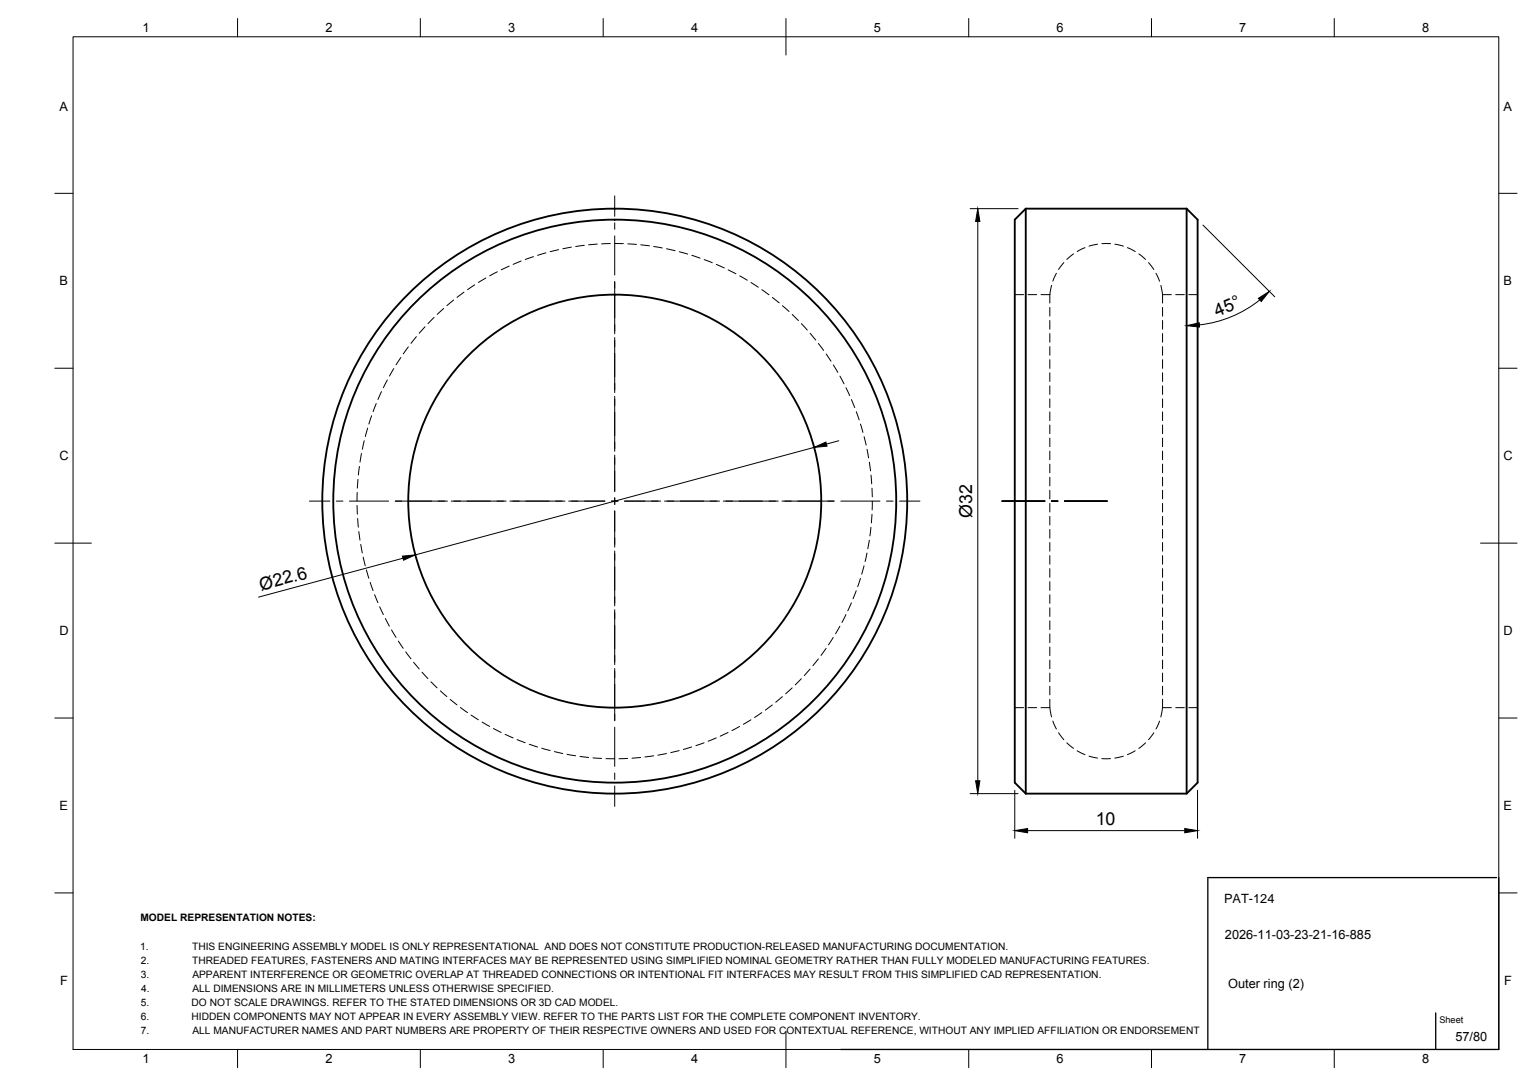
ISO-10303-21;
HEADER;
/* Generated by software containing ST-Developer
 * from STEP Tools, Inc. (www.steptools.com) 
 */

FILE_DESCRIPTION(
/* description */ ('XY cross-slide table'),
/* implementation_level */ '2;1');

FILE_NAME(
/* name */ 'Outer ring (2).step',
/* time_stamp */ '2026-10-28T03:22:46-07:00',
/* author */ (''),
/* organization */ (''),
/* preprocessor_version */ 'ST-DEVELOPER v20.2',
/* originating_system */ 'Autodesk Translation Framework v15.17.0.0',
/* authorisation */ '');

FILE_SCHEMA (('AUTOMOTIVE_DESIGN { 1 0 10303 214 3 1 1 }'));
ENDSEC;

DATA;
#10=MECHANICAL_DESIGN_GEOMETRIC_PRESENTATION_REPRESENTATION('',(#1737),#62984);
#1469=CONICAL_SURFACE('',#25563,1.57,0.785398163397449);
#1470=CONICAL_SURFACE('',#25567,1.57,0.785398163397449);
#1501=TOROIDAL_SURFACE('',#25552,1.1,0.309556);
#1556=SHAPE_REPRESENTATION_RELATIONSHIP('SRR','None',#63412,#1639);
#1639=ADVANCED_BREP_SHAPE_REPRESENTATION('',(#1846),#62949);
#1737=STYLED_ITEM('',(#63912),#1846);
#1846=MANIFOLD_SOLID_BREP('Body1',#23035);
#2203=FACE_BOUND('',#5316,.T.);
#2204=FACE_BOUND('',#5321,.T.);
#2664=PLANE('',#25560);
#2665=PLANE('',#25569);
#3683=FACE_OUTER_BOUND('',#5313,.T.);
#3684=FACE_OUTER_BOUND('',#5314,.T.);
#3685=FACE_OUTER_BOUND('',#5315,.T.);
#3686=FACE_OUTER_BOUND('',#5317,.T.);
#3687=FACE_OUTER_BOUND('',#5318,.T.);
#3688=FACE_OUTER_BOUND('',#5319,.T.);
#3689=FACE_OUTER_BOUND('',#5320,.T.);
#3690=FACE_OUTER_BOUND('',#5322,.T.);
#5313=EDGE_LOOP('',(#18660,#18661,#18662,#18663,#18664,#18665));
#5314=EDGE_LOOP('',(#18666,#18667,#18668,#18669,#18670));
#5315=EDGE_LOOP('',(#18671));
#5316=EDGE_LOOP('',(#18672));
#5317=EDGE_LOOP('',(#18673,#18674,#18675,#18676));
#5318=EDGE_LOOP('',(#18677,#18678,#18679,#18680));
#5319=EDGE_LOOP('',(#18681,#18682,#18683,#18684));
#5320=EDGE_LOOP('',(#18685));
#5321=EDGE_LOOP('',(#18686));
#5322=EDGE_LOOP('',(#18687,#18688,#18689,#18690,#18691));
#6842=LINE('',#48582,#8329);
#6843=LINE('',#48591,#8330);
#6844=LINE('',#48595,#8331);
#6845=LINE('',#48599,#8332);
#6846=LINE('',#48602,#8333);
#8329=VECTOR('',#30517,1.129765);
#8330=VECTOR('',#30528,1.57);
#8331=VECTOR('',#30533,1.6);
#8332=VECTOR('',#30538,1.57);
#8333=VECTOR('',#30543,1.129765);
#9478=CIRCLE('',#25553,1.129765);
#9479=CIRCLE('',#25554,1.129765);
#9480=CIRCLE('',#25555,0.309556);
#9481=CIRCLE('',#25556,1.129765);
#9482=CIRCLE('',#25557,1.129765);
#9483=CIRCLE('',#25559,1.129765);
#9484=CIRCLE('',#25561,1.54);
#9485=CIRCLE('',#25562,1.129765);
#9486=CIRCLE('',#25564,1.6);
#9487=CIRCLE('',#25566,1.6);
#9488=CIRCLE('',#25568,1.54);
#11031=VERTEX_POINT('',#48570);
#11032=VERTEX_POINT('',#48571);
#11033=VERTEX_POINT('',#48574);
#11034=VERTEX_POINT('',#48576);
#11035=VERTEX_POINT('',#48580);
#11036=VERTEX_POINT('',#48584);
#11037=VERTEX_POINT('',#48586);
#11038=VERTEX_POINT('',#48589);
#11039=VERTEX_POINT('',#48593);
#11040=VERTEX_POINT('',#48597);
#13714=EDGE_CURVE('',#11031,#11032,#9478,.T.);
#13715=EDGE_CURVE('',#11032,#11031,#9479,.T.);
#13716=EDGE_CURVE('',#11032,#11033,#9480,.T.);
#13717=EDGE_CURVE('',#11034,#11033,#9481,.T.);
#13718=EDGE_CURVE('',#11033,#11034,#9482,.T.);
#13719=EDGE_CURVE('',#11035,#11035,#9483,.T.);
#13720=EDGE_CURVE('',#11035,#11034,#6842,.T.);
#13721=EDGE_CURVE('',#11036,#11036,#9484,.T.);
#13722=EDGE_CURVE('',#11037,#11037,#9485,.T.);
#13723=EDGE_CURVE('',#11038,#11038,#9486,.T.);
#13724=EDGE_CURVE('',#11038,#11036,#6843,.T.);
#13725=EDGE_CURVE('',#11039,#11039,#9487,.T.);
#13726=EDGE_CURVE('',#11039,#11038,#6844,.T.);
#13727=EDGE_CURVE('',#11040,#11040,#9488,.T.);
#13728=EDGE_CURVE('',#11040,#11039,#6845,.T.);
#13729=EDGE_CURVE('',#11031,#11037,#6846,.T.);
#18660=ORIENTED_EDGE('',*,*,#13714,.F.);
#18661=ORIENTED_EDGE('',*,*,#13715,.F.);
#18662=ORIENTED_EDGE('',*,*,#13716,.T.);
#18663=ORIENTED_EDGE('',*,*,#13717,.F.);
#18664=ORIENTED_EDGE('',*,*,#13718,.F.);
#18665=ORIENTED_EDGE('',*,*,#13716,.F.);
#18666=ORIENTED_EDGE('',*,*,#13719,.T.);
#18667=ORIENTED_EDGE('',*,*,#13720,.T.);
#18668=ORIENTED_EDGE('',*,*,#13717,.T.);
#18669=ORIENTED_EDGE('',*,*,#13718,.T.);
#18670=ORIENTED_EDGE('',*,*,#13720,.F.);
#18671=ORIENTED_EDGE('',*,*,#13721,.F.);
#18672=ORIENTED_EDGE('',*,*,#13722,.T.);
#18673=ORIENTED_EDGE('',*,*,#13723,.F.);
#18674=ORIENTED_EDGE('',*,*,#13724,.T.);
#18675=ORIENTED_EDGE('',*,*,#13721,.T.);
#18676=ORIENTED_EDGE('',*,*,#13724,.F.);
#18677=ORIENTED_EDGE('',*,*,#13725,.F.);
#18678=ORIENTED_EDGE('',*,*,#13726,.T.);
#18679=ORIENTED_EDGE('',*,*,#13723,.T.);
#18680=ORIENTED_EDGE('',*,*,#13726,.F.);
#18681=ORIENTED_EDGE('',*,*,#13727,.F.);
#18682=ORIENTED_EDGE('',*,*,#13728,.T.);
#18683=ORIENTED_EDGE('',*,*,#13725,.T.);
#18684=ORIENTED_EDGE('',*,*,#13728,.F.);
#18685=ORIENTED_EDGE('',*,*,#13727,.T.);
#18686=ORIENTED_EDGE('',*,*,#13719,.F.);
#18687=ORIENTED_EDGE('',*,*,#13714,.T.);
#18688=ORIENTED_EDGE('',*,*,#13715,.T.);
#18689=ORIENTED_EDGE('',*,*,#13729,.T.);
#18690=ORIENTED_EDGE('',*,*,#13722,.F.);
#18691=ORIENTED_EDGE('',*,*,#13729,.F.);
#21419=CYLINDRICAL_SURFACE('',#25558,1.129765);
#21420=CYLINDRICAL_SURFACE('',#25565,1.6);
#21421=CYLINDRICAL_SURFACE('',#25570,1.129765);
#22464=ADVANCED_FACE('',(#3683),#1501,.F.);
#22465=ADVANCED_FACE('',(#3684),#21419,.F.);
#22466=ADVANCED_FACE('',(#3685,#2203),#2664,.T.);
#22467=ADVANCED_FACE('',(#3686),#1469,.T.);
#22468=ADVANCED_FACE('',(#3687),#21420,.T.);
#22469=ADVANCED_FACE('',(#3688),#1470,.T.);
#22470=ADVANCED_FACE('',(#3689,#2204),#2665,.T.);
#22471=ADVANCED_FACE('',(#3690),#21421,.F.);
#23035=CLOSED_SHELL('',(#22464,#22465,#22466,#22467,#22468,#22469,#22470,
#22471));
#25551=AXIS2_PLACEMENT_3D('',#48568,#30499,#30500);
#25552=AXIS2_PLACEMENT_3D('',#48569,#30501,#30502);
#25553=AXIS2_PLACEMENT_3D('',#48572,#30503,#30504);
#25554=AXIS2_PLACEMENT_3D('',#48573,#30505,#30506);
#25555=AXIS2_PLACEMENT_3D('',#48575,#30507,#30508);
#25556=AXIS2_PLACEMENT_3D('',#48577,#30509,#30510);
#25557=AXIS2_PLACEMENT_3D('',#48578,#30511,#30512);
#25558=AXIS2_PLACEMENT_3D('',#48579,#30513,#30514);
#25559=AXIS2_PLACEMENT_3D('',#48581,#30515,#30516);
#25560=AXIS2_PLACEMENT_3D('',#48583,#30518,#30519);
#25561=AXIS2_PLACEMENT_3D('',#48585,#30520,#30521);
#25562=AXIS2_PLACEMENT_3D('',#48587,#30522,#30523);
#25563=AXIS2_PLACEMENT_3D('',#48588,#30524,#30525);
#25564=AXIS2_PLACEMENT_3D('',#48590,#30526,#30527);
#25565=AXIS2_PLACEMENT_3D('',#48592,#30529,#30530);
#25566=AXIS2_PLACEMENT_3D('',#48594,#30531,#30532);
#25567=AXIS2_PLACEMENT_3D('',#48596,#30534,#30535);
#25568=AXIS2_PLACEMENT_3D('',#48598,#30536,#30537);
#25569=AXIS2_PLACEMENT_3D('',#48600,#30539,#30540);
#25570=AXIS2_PLACEMENT_3D('',#48601,#30541,#30542);
#30499=DIRECTION('axis',(0.,0.,1.));
#30500=DIRECTION('refdir',(1.,0.,0.));
#30501=DIRECTION('center_axis',(0.,-1.,0.));
#30502=DIRECTION('ref_axis',(0.,0.,-1.));
#30503=DIRECTION('center_axis',(0.,-1.,0.));
#30504=DIRECTION('ref_axis',(1.,0.,0.));
#30505=DIRECTION('center_axis',(0.,-1.,0.));
#30506=DIRECTION('ref_axis',(1.,0.,0.));
#30507=DIRECTION('center_axis',(1.,0.,1.22464679914735E-16));
#30508=DIRECTION('ref_axis',(-1.22464679914735E-16,0.,1.));
#30509=DIRECTION('center_axis',(0.,1.,0.));
#30510=DIRECTION('ref_axis',(1.,0.,0.));
#30511=DIRECTION('center_axis',(0.,1.,0.));
#30512=DIRECTION('ref_axis',(1.,0.,0.));
#30513=DIRECTION('center_axis',(0.,-1.,0.));
#30514=DIRECTION('ref_axis',(1.,0.,0.));
#30515=DIRECTION('center_axis',(0.,-1.,0.));
#30516=DIRECTION('ref_axis',(1.,0.,0.));
#30517=DIRECTION('',(0.,1.,0.));
#30518=DIRECTION('center_axis',(0.,1.,0.));
#30519=DIRECTION('ref_axis',(0.,0.,1.));
#30520=DIRECTION('center_axis',(0.,-1.,0.));
#30521=DIRECTION('ref_axis',(1.,0.,0.));
#30522=DIRECTION('center_axis',(0.,-1.,0.));
#30523=DIRECTION('ref_axis',(1.,0.,0.));
#30524=DIRECTION('center_axis',(0.,-1.,0.));
#30525=DIRECTION('ref_axis',(1.,0.,0.));
#30526=DIRECTION('center_axis',(0.,-1.,0.));
#30527=DIRECTION('ref_axis',(1.,0.,0.));
#30528=DIRECTION('',(0.707106781186548,0.707106781186547,8.65956056235494E-17));
#30529=DIRECTION('center_axis',(0.,-1.,0.));
#30530=DIRECTION('ref_axis',(1.,0.,0.));
#30531=DIRECTION('center_axis',(0.,-1.,0.));
#30532=DIRECTION('ref_axis',(1.,0.,0.));
#30533=DIRECTION('',(0.,1.,0.));
#30534=DIRECTION('center_axis',(0.,1.,0.));
#30535=DIRECTION('ref_axis',(1.,0.,0.));
#30536=DIRECTION('center_axis',(0.,-1.,0.));
#30537=DIRECTION('ref_axis',(1.,0.,0.));
#30538=DIRECTION('',(-0.707106781186548,0.707106781186547,-8.65956056235494E-17));
#30539=DIRECTION('center_axis',(0.,-1.,0.));
#30540=DIRECTION('ref_axis',(0.,0.,-1.));
#30541=DIRECTION('center_axis',(0.,-1.,0.));
#30542=DIRECTION('ref_axis',(1.,0.,0.));
#30543=DIRECTION('',(0.,1.,0.));
#48568=CARTESIAN_POINT('',(0.,0.,0.));
#48569=CARTESIAN_POINT('Origin',(0.,0.,0.));
#48570=CARTESIAN_POINT('',(-1.129765,0.308121667383195,-1.38356309103871E-16));
#48571=CARTESIAN_POINT('',(-1.38356309103871E-16,0.308121667383195,1.129765));
#48572=CARTESIAN_POINT('Origin',(0.,0.308121667383195,0.));
#48573=CARTESIAN_POINT('Origin',(0.,0.308121667383195,0.));
#48574=CARTESIAN_POINT('',(-1.38356309103871E-16,-0.308121667383195,1.129765));
#48575=CARTESIAN_POINT('Origin',(-1.34711147906209E-16,0.,1.1));
#48576=CARTESIAN_POINT('',(-1.129765,-0.308121667383195,1.38356309103871E-16));
#48577=CARTESIAN_POINT('Origin',(0.,-0.308121667383195,0.));
#48578=CARTESIAN_POINT('Origin',(0.,-0.308121667383195,0.));
#48579=CARTESIAN_POINT('Origin',(0.,0.,0.));
#48580=CARTESIAN_POINT('',(-1.129765,-0.5,-1.38356309103871E-16));
#48581=CARTESIAN_POINT('Origin',(0.,-0.5,0.));
#48582=CARTESIAN_POINT('',(-1.129765,0.,-1.38356309103871E-16));
#48583=CARTESIAN_POINT('Origin',(1.54,0.5,0.));
#48584=CARTESIAN_POINT('',(-1.54,0.5,-1.88595607068692E-16));
#48585=CARTESIAN_POINT('Origin',(0.,0.5,0.));
#48586=CARTESIAN_POINT('',(-1.129765,0.5,-1.38356309103871E-16));
#48587=CARTESIAN_POINT('Origin',(0.,0.5,0.));
#48588=CARTESIAN_POINT('Origin',(0.,0.47,0.));
#48589=CARTESIAN_POINT('',(-1.6,0.44,-1.95943487863577E-16));
#48590=CARTESIAN_POINT('Origin',(0.,0.44,0.));
#48591=CARTESIAN_POINT('',(-1.57,0.47,-1.92269547466134E-16));
#48592=CARTESIAN_POINT('Origin',(0.,0.,0.));
#48593=CARTESIAN_POINT('',(-1.6,-0.44,-1.95943487863577E-16));
#48594=CARTESIAN_POINT('Origin',(0.,-0.44,0.));
#48595=CARTESIAN_POINT('',(-1.6,0.,-1.95943487863577E-16));
#48596=CARTESIAN_POINT('Origin',(0.,-0.47,0.));
#48597=CARTESIAN_POINT('',(-1.54,-0.5,-1.88595607068692E-16));
#48598=CARTESIAN_POINT('Origin',(0.,-0.5,0.));
#48599=CARTESIAN_POINT('',(-1.57,-0.47,-1.92269547466134E-16));
#48600=CARTESIAN_POINT('Origin',(1.129765,-0.5,0.));
#48601=CARTESIAN_POINT('Origin',(0.,0.,0.));
#48602=CARTESIAN_POINT('',(-1.129765,0.,-1.38356309103871E-16));
#62850=UNCERTAINTY_MEASURE_WITH_UNIT(LENGTH_MEASURE(0.001),#62985,
'DISTANCE_ACCURACY_VALUE',
'Maximum model space distance between geometric entities at asserted c
onnectivities');
#62885=UNCERTAINTY_MEASURE_WITH_UNIT(LENGTH_MEASURE(0.001),#62985,
'DISTANCE_ACCURACY_VALUE',
'Maximum model space distance between geometric entities at asserted c
onnectivities');
#62949=(
GEOMETRIC_REPRESENTATION_CONTEXT(3)
GLOBAL_UNCERTAINTY_ASSIGNED_CONTEXT((#62850))
GLOBAL_UNIT_ASSIGNED_CONTEXT((#62985,#62987,#62988))
REPRESENTATION_CONTEXT('','3D')
);
#62984=(
GEOMETRIC_REPRESENTATION_CONTEXT(3)
GLOBAL_UNCERTAINTY_ASSIGNED_CONTEXT((#62885))
GLOBAL_UNIT_ASSIGNED_CONTEXT((#62985,#62987,#62988))
REPRESENTATION_CONTEXT('','3D')
);
#62985=(
LENGTH_UNIT()
NAMED_UNIT(*)
SI_UNIT(.CENTI.,.METRE.)
);
#62987=(
NAMED_UNIT(*)
PLANE_ANGLE_UNIT()
SI_UNIT($,.RADIAN.)
);
#62988=(
NAMED_UNIT(*)
SI_UNIT($,.STERADIAN.)
SOLID_ANGLE_UNIT()
);
#63052=SHAPE_DEFINITION_REPRESENTATION(#63230,#63412);
#63230=PRODUCT_DEFINITION_SHAPE('',$,#63511);
#63412=SHAPE_REPRESENTATION('',(#25551),#62949);
#63447=PRODUCT_DEFINITION_CONTEXT('part definition',#63743,'design');
#63511=PRODUCT_DEFINITION('Outer ring (2)','Outer ring (2)',#63609,#63447);
#63609=PRODUCT_DEFINITION_FORMATION('',$,#63808);
#63743=APPLICATION_CONTEXT(
'Core Data for Automotive Mechanical Design Process');
#63744=PRODUCT_CONTEXT('part definition',#63743,'mechanical');
#63808=PRODUCT('Outer ring (2)','Outer ring (2)','Outer ring (2)',(#63744));
#63906=COLOUR_RGB('Grey',0.48,0.52,0.57);
#63907=FILL_AREA_STYLE_COLOUR('',#63906);
#63908=FILL_AREA_STYLE('',(#63907));
#63909=SURFACE_STYLE_FILL_AREA(#63908);
#63910=SURFACE_SIDE_STYLE('',(#63909));
#63911=SURFACE_STYLE_USAGE(.BOTH.,#63910);
#63912=PRESENTATION_STYLE_ASSIGNMENT((#63911));
ENDSEC;
END-ISO-10303-21;
